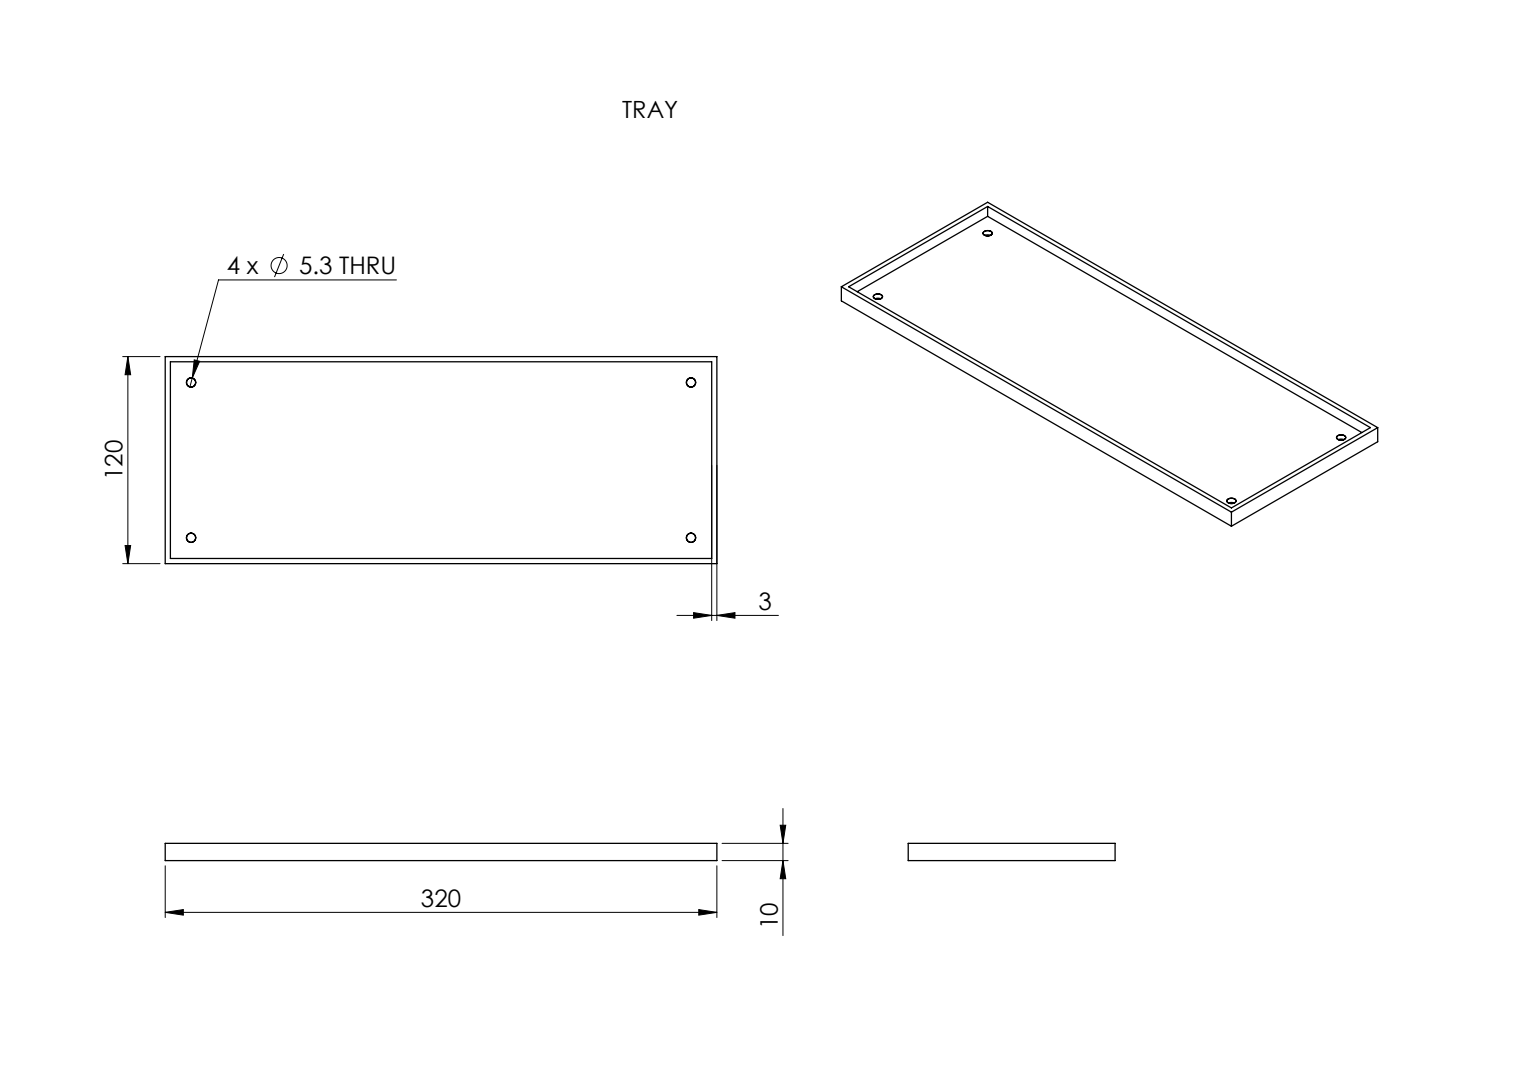
ISO-10303-21;
HEADER;
FILE_DESCRIPTION (('STEP AP214'),
    '1' );
FILE_NAME ('tray.step',
    '2026-10-23T15:04:32',
    ( '' ),
    ( '' ),
    'SwSTEP 2.0',
    'SolidWorks 2026',
    '' );
FILE_SCHEMA (( 'AUTOMOTIVE_DESIGN' ));
ENDSEC;

DATA;
#6=ORIENTED_EDGE ( 'NONE', *, *, #567, .F. ) ;
#7=CARTESIAN_POINT ( 'NONE',  ( 145.0000000000000284, 2.993649167310367343, -47.64999999999998437 ) ) ;
#14=ORIENTED_EDGE ( 'NONE', *, *, #1898, .T. ) ;
#15=FACE_OUTER_BOUND ( 'NONE', #510, .T. ) ;
#18=CIRCLE ( 'NONE', #321, 2.700000000000001066 ) ;
#19=ORIENTED_EDGE ( 'NONE', *, *, #1395, .T. ) ;
#21=CARTESIAN_POINT ( 'NONE',  ( 157.0000000000000000, 10.00000000000000000, 3.631354476378115974E-14 ) ) ;
#24=ORIENTED_EDGE ( 'NONE', *, *, #1544, .T. ) ;
#25=CARTESIAN_POINT ( 'NONE',  ( -145.0000000000000284, 3.000000000000000000, -45.00000000000000000 ) ) ;
#26=DIRECTION ( 'NONE',  ( -0.000000000000000000, 1.000000000000000000, -0.000000000000000000 ) ) ;
#27=CYLINDRICAL_SURFACE ( 'NONE', #1694, 2.649999999999985700 ) ;
#30=AXIS2_PLACEMENT_3D ( 'NONE', #971, #1660, #79 ) ;
#31=CIRCLE ( 'NONE', #984, 2.649999999999985700 ) ;
#35=ORIENTED_EDGE ( 'NONE', *, *, #686, .F. ) ;
#36=CYLINDRICAL_SURFACE ( 'NONE', #640, 2.649999999999985700 ) ;
#39=DIRECTION ( 'NONE',  ( -6.123233995736766036E-17, 1.000000000000000000, -0.000000000000000000 ) ) ;
#44=VERTEX_POINT ( 'NONE', #1009 ) ;
#46=CARTESIAN_POINT ( 'NONE',  ( 160.0000000000000000, 0.000000000000000000, -60.00000000000000000 ) ) ;
#47=CARTESIAN_POINT ( 'NONE',  ( 160.0000000000000000, 10.00000000000000000, -60.00000000000000000 ) ) ;
#48=PLANE ( 'NONE',  #876 ) ;
#49=ORIENTED_EDGE ( 'NONE', *, *, #111, .T. ) ;
#50=DIRECTION ( 'NONE',  ( -0.000000000000000000, 1.000000000000000000, -0.000000000000000000 ) ) ;
#51=AXIS2_PLACEMENT_3D ( 'NONE', #1269, #57, #1759 ) ;
#57=DIRECTION ( 'NONE',  ( 6.123233995736766036E-17, -1.000000000000000000, 0.000000000000000000 ) ) ;
#59=DIRECTION ( 'NONE',  ( -0.000000000000000000, -1.000000000000000000, -0.000000000000000000 ) ) ;
#60=VERTEX_POINT ( 'NONE', #817 ) ;
#66=ADVANCED_FACE ( 'NONE', ( #1330, #2016 ), #1163, .F. ) ;
#67=AXIS2_PLACEMENT_3D ( 'NONE', #1690, #1835, #1322 ) ;
#69=DIRECTION ( 'NONE',  ( -1.000000000000000000, 0.000000000000000000, -0.000000000000000000 ) ) ;
#70=LINE ( 'NONE', #2132, #1985 ) ;
#71=AXIS2_PLACEMENT_3D ( 'NONE', #2013, #995, #1317 ) ;
#73=CARTESIAN_POINT ( 'NONE',  ( 145.0000000000000284, 2.993649167310367343, -45.00000000000000000 ) ) ;
#77=DIRECTION ( 'NONE',  ( 0.000000000000000000, 0.000000000000000000, -1.000000000000000000 ) ) ;
#79=DIRECTION ( 'NONE',  ( 1.000000000000000000, 0.000000000000000000, 0.000000000000000000 ) ) ;
#82=FACE_OUTER_BOUND ( 'NONE', #1924, .T. ) ;
#88=VECTOR ( 'NONE', #539, 1000.000000000000000 ) ;
#90=CARTESIAN_POINT ( 'NONE',  ( -157.0000000000000284, 10.00000000000000000, 57.00000000000000711 ) ) ;
#93=( LENGTH_UNIT ( ) NAMED_UNIT ( * ) SI_UNIT ( .MILLI., .METRE. ) );
#100=ORIENTED_EDGE ( 'NONE', *, *, #520, .T. ) ;
#102=CARTESIAN_POINT ( 'NONE',  ( -160.0000000000000000, 10.00000000000000000, -56.99999999999997868 ) ) ;
#103=AXIS2_PLACEMENT_3D ( 'NONE', #1867, #1367, #311 ) ;
#109=PLANE ( 'NONE',  #1726 ) ;
#111=EDGE_CURVE ( 'NONE', #1963, #60, #1752, .T. ) ;
#114=DIRECTION ( 'NONE',  ( 1.000000000000000000, 0.000000000000000000, -4.336808689942017736E-17 ) ) ;
#117=( GEOMETRIC_REPRESENTATION_CONTEXT ( 3 ) GLOBAL_UNCERTAINTY_ASSIGNED_CONTEXT ( ( #842 ) ) GLOBAL_UNIT_ASSIGNED_CONTEXT ( ( #1606, #589, #1445 ) ) REPRESENTATION_CONTEXT ( 'NONE', 'WORKASPACE' ) );
#119=CARTESIAN_POINT ( 'NONE',  ( -145.0000000000000284, 0.000000000000000000, 42.35000000000001563 ) ) ;
#120=CARTESIAN_POINT ( 'NONE',  ( 156.9999999999999716, 3.000000000000000000, 57.00000000000000711 ) ) ;
#121=EDGE_CURVE ( 'NONE', #1963, #166, #205, .T. ) ;
#128=DIRECTION ( 'NONE',  ( 1.000000000000000000, 0.000000000000000000, 0.000000000000000000 ) ) ;
#129=AXIS2_PLACEMENT_3D ( 'NONE', #1889, #358, #1728 ) ;
#131=FILL_AREA_STYLE_COLOUR ( '', #721 ) ;
#135=EDGE_CURVE ( 'NONE', #1670, #1316, #2046, .T. ) ;
#137=CARTESIAN_POINT ( 'NONE',  ( 145.0000000000000284, 3.000000000000002665, -45.00000000000000000 ) ) ;
#142=DIRECTION ( 'NONE',  ( 0.000000000000000000, 0.000000000000000000, -1.000000000000000000 ) ) ;
#146=ADVANCED_FACE ( 'NONE', ( #978 ), #2193, .F. ) ;
#148=ORIENTED_EDGE ( 'NONE', *, *, #1970, .F. ) ;
#151=ORIENTED_EDGE ( 'NONE', *, *, #1176, .T. ) ;
#152=VECTOR ( 'NONE', #723, 1000.000000000000000 ) ;
#154=FACE_OUTER_BOUND ( 'NONE', #1037, .T. ) ;
#158=ORIENTED_EDGE ( 'NONE', *, *, #281, .T. ) ;
#159=DIRECTION ( 'NONE',  ( 0.000000000000000000, -1.000000000000000000, 0.000000000000000000 ) ) ;
#160=CARTESIAN_POINT ( 'NONE',  ( -145.0000000000000284, 3.000000000000001776, -47.70000000000000284 ) ) ;
#166=VERTEX_POINT ( 'NONE', #1403 ) ;
#167=ORIENTED_EDGE ( 'NONE', *, *, #1762, .T. ) ;
#168=VECTOR ( 'NONE', #1538, 1000.000000000000000 ) ;
#169=CYLINDRICAL_SURFACE ( 'NONE', #1242, 2.649999999999985700 ) ;
#170=CARTESIAN_POINT ( 'NONE',  ( -157.0000000000000000, 10.00000000000000000, -3.631354476378115974E-14 ) ) ;
#171=ADVANCED_FACE ( 'NONE', ( #512 ), #704, .T. ) ;
#176=ORIENTED_EDGE ( 'NONE', *, *, #1772, .T. ) ;
#177=AXIS2_PLACEMENT_3D ( 'NONE', #1608, #438, #449 ) ;
#178=ORIENTED_EDGE ( 'NONE', *, *, #684, .F. ) ;
#179=FACE_OUTER_BOUND ( 'NONE', #272, .T. ) ;
#181=CARTESIAN_POINT ( 'NONE',  ( -160.0000000000000284, 0.000000000000000000, 60.00000000000001421 ) ) ;
#182=AXIS2_PLACEMENT_3D ( 'NONE', #632, #455, #1006 ) ;
#186=EDGE_CURVE ( 'NONE', #1465, #166, #1054, .T. ) ;
#197=EDGE_CURVE ( 'NONE', #1465, #610, #889, .T. ) ;
#199=LINE ( 'NONE', #1861, #548 ) ;
#202=CARTESIAN_POINT ( 'NONE',  ( 145.0000000000000284, 3.000000000000001776, -47.70000000000000284 ) ) ;
#204=ORIENTED_EDGE ( 'NONE', *, *, #1315, .F. ) ;
#205=CIRCLE ( 'NONE', #1463, 2.649999999999985700 ) ;
#210=CARTESIAN_POINT ( 'NONE',  ( -160.0000000000000000, 10.00000000000000000, -59.99999999999998579 ) ) ;
#211=DIRECTION ( 'NONE',  ( 0.000000000000000000, 0.000000000000000000, -1.000000000000000000 ) ) ;
#214=EDGE_LOOP ( 'NONE', ( #762, #945, #1306, #1209 ) ) ;
#216=VERTEX_POINT ( 'NONE', #7 ) ;
#217=FACE_OUTER_BOUND ( 'NONE', #1185, .T. ) ;
#218=CARTESIAN_POINT ( 'NONE',  ( 160.0000000000000000, 10.00000000000000000, -60.00000000000000000 ) ) ;
#219=DIRECTION ( 'NONE',  ( 4.336808689942017736E-17, -0.000000000000000000, 1.000000000000000000 ) ) ;
#223=DIRECTION ( 'NONE',  ( -1.000000000000000000, -6.123233995736766036E-17, -0.000000000000000000 ) ) ;
#225=ORIENTED_EDGE ( 'NONE', *, *, #1492, .F. ) ;
#227=CIRCLE ( 'NONE', #385, 2.700000000000001066 ) ;
#230=CARTESIAN_POINT ( 'NONE',  ( -160.0000000000000284, 10.00000000000000000, 60.00000000000001421 ) ) ;
#231=CARTESIAN_POINT ( 'NONE',  ( -2.471980953266949321E-15, 3.000000000000000000, -56.99999999999998579 ) ) ;
#234=ORIENTED_EDGE ( 'NONE', *, *, #1075, .T. ) ;
#235=ORIENTED_EDGE ( 'NONE', *, *, #197, .F. ) ;
#238=FACE_OUTER_BOUND ( 'NONE', #1600, .T. ) ;
#240=VERTEX_POINT ( 'NONE', #1377 ) ;
#242=AXIS2_PLACEMENT_3D ( 'NONE', #919, #223, #2104 ) ;
#243=DIRECTION ( 'NONE',  ( -1.000000000000000000, 0.000000000000000000, 4.336808689942017736E-17 ) ) ;
#246=ADVANCED_FACE ( 'NONE', ( #1385 ), #1674, .T. ) ;
#250=VECTOR ( 'NONE', #1166, 1000.000000000000000 ) ;
#251=ORIENTED_EDGE ( 'NONE', *, *, #1272, .F. ) ;
#252=DIRECTION ( 'NONE',  ( -0.000000000000000000, 1.000000000000000000, -0.000000000000000000 ) ) ;
#253=CARTESIAN_POINT ( 'NONE',  ( -145.0000000000000284, 3.000000000000002665, 45.00000000000000000 ) ) ;
#256=VERTEX_POINT ( 'NONE', #1555 ) ;
#258=DIRECTION ( 'NONE',  ( -0.000000000000000000, 1.000000000000000000, -0.000000000000000000 ) ) ;
#259=ORIENTED_EDGE ( 'NONE', *, *, #781, .F. ) ;
#260=DIRECTION ( 'NONE',  ( -1.000000000000000000, -6.123233995736766036E-17, -0.000000000000000000 ) ) ;
#261=SHAPE_REPRESENTATION ( 'tray', ( #30 ), #1049 ) ;
#262=DIRECTION ( 'NONE',  ( 0.000000000000000000, -1.000000000000000000, 0.000000000000000000 ) ) ;
#263=LINE ( 'NONE', #90, #1184 ) ;
#266=EDGE_CURVE ( 'NONE', #1421, #653, #1916, .T. ) ;
#267=VERTEX_POINT ( 'NONE', #707 ) ;
#272=EDGE_LOOP ( 'NONE', ( #1135, #854, #1328, #1129 ) ) ;
#273=CARTESIAN_POINT ( 'NONE',  ( 145.0000000000000284, 2.800000000000000266, -45.00000000000000000 ) ) ;
#276=FACE_OUTER_BOUND ( 'NONE', #1110, .T. ) ;
#279=PRODUCT_DEFINITION_SHAPE ( 'NONE', 'NONE',  #1642 ) ;
#281=EDGE_CURVE ( 'NONE', #240, #1735, #1638, .T. ) ;
#282=ORIENTED_EDGE ( 'NONE', *, *, #559, .F. ) ;
#287=ADVANCED_FACE ( 'NONE', ( #15 ), #36, .F. ) ;
#298=AXIS2_PLACEMENT_3D ( 'NONE', #2174, #1189, #2020 ) ;
#305=ADVANCED_FACE ( 'NONE', ( #1736 ), #169, .F. ) ;
#307=( NAMED_UNIT ( * ) PLANE_ANGLE_UNIT ( ) SI_UNIT ( $, .RADIAN. ) );
#308=ORIENTED_EDGE ( 'NONE', *, *, #734, .F. ) ;
#311=DIRECTION ( 'NONE',  ( 0.000000000000000000, -1.000000000000000000, 0.000000000000000000 ) ) ;
#315=DIRECTION ( 'NONE',  ( -6.123233995736766036E-17, 1.000000000000000000, -0.000000000000000000 ) ) ;
#317=CARTESIAN_POINT ( 'NONE',  ( -145.0000000000000284, 0.000000000000000000, -45.00000000000000000 ) ) ;
#321=AXIS2_PLACEMENT_3D ( 'NONE', #1424, #399, #1951 ) ;
#323=DIRECTION ( 'NONE',  ( -0.000000000000000000, 1.000000000000000000, -0.000000000000000000 ) ) ;
#326=DIRECTION ( 'NONE',  ( 6.123233995736766036E-17, -1.000000000000000000, 0.000000000000000000 ) ) ;
#330=DIRECTION ( 'NONE',  ( 2.312964634635742957E-16, 0.000000000000000000, -1.000000000000000000 ) ) ;
#332=ORIENTED_EDGE ( 'NONE', *, *, #1547, .T. ) ;
#334=EDGE_CURVE ( 'NONE', #396, #60, #18, .T. ) ;
#336=MECHANICAL_DESIGN_GEOMETRIC_PRESENTATION_REPRESENTATION('',(#1119),#1476);
#337=ORIENTED_EDGE ( 'NONE', *, *, #2208, .F. ) ;
#339=CARTESIAN_POINT ( 'NONE',  ( -157.0000000000000284, 3.000000000000000000, 57.00000000000000711 ) ) ;
#341=STYLED_ITEM('',(#2247),#969);
#343=EDGE_LOOP ( 'NONE', ( #996, #736, #151, #176 ) ) ;
#344=VERTEX_POINT ( 'NONE', #572 ) ;
#345=ADVANCED_FACE ( 'NONE', ( #1256 ), #564, .T. ) ;
#346=DIRECTION ( 'NONE',  ( 0.000000000000000000, 0.000000000000000000, 1.000000000000000000 ) ) ;
#348=UNCERTAINTY_MEASURE_WITH_UNIT (LENGTH_MEASURE( 1.000000000000000082E-05 ), #93, 'distance_accuracy_value', 'NONE');
#350=DIRECTION ( 'NONE',  ( 1.000000000000000000, 0.000000000000000000, 0.000000000000000000 ) ) ;
#351=EDGE_LOOP ( 'NONE', ( #436, #2147 ) ) ;
#352=ADVANCED_FACE ( 'NONE', ( #217 ), #1742, .T. ) ;
#353=VERTEX_POINT ( 'NONE', #46 ) ;
#355=AXIS2_PLACEMENT_3D ( 'NONE', #1066, #872, #1906 ) ;
#358=DIRECTION ( 'NONE',  ( 6.123233995736766036E-17, -1.000000000000000000, 0.000000000000000000 ) ) ;
#365=DIRECTION ( 'NONE',  ( 0.000000000000000000, 0.000000000000000000, -1.000000000000000000 ) ) ;
#375=EDGE_LOOP ( 'NONE', ( #1502, #922, #259, #2033 ) ) ;
#377=DIRECTION ( 'NONE',  ( 0.000000000000000000, -1.000000000000000000, 0.000000000000000000 ) ) ;
#379=EDGE_LOOP ( 'NONE', ( #1466, #491 ) ) ;
#381=EDGE_CURVE ( 'NONE', #344, #473, #457, .T. ) ;
#385=AXIS2_PLACEMENT_3D ( 'NONE', #1320, #1495, #1483 ) ;
#386=ORIENTED_EDGE ( 'NONE', *, *, #744, .T. ) ;
#387=ORIENTED_EDGE ( 'NONE', *, *, #767, .F. ) ;
#389=CYLINDRICAL_SURFACE ( 'NONE', #1669, 2.649999999999985700 ) ;
#390=PLANE ( 'NONE',  #760 ) ;
#392=CARTESIAN_POINT ( 'NONE',  ( -160.0000000000000284, 10.00000000000000000, 60.00000000000001421 ) ) ;
#396=VERTEX_POINT ( 'NONE', #2094 ) ;
#397=VECTOR ( 'NONE', #1100, 1000.000000000000000 ) ;
#399=DIRECTION ( 'NONE',  ( -6.123233995736766036E-17, 1.000000000000000000, -0.000000000000000000 ) ) ;
#408=DIRECTION ( 'NONE',  ( 0.000000000000000000, 0.000000000000000000, -1.000000000000000000 ) ) ;
#409=DIRECTION ( 'NONE',  ( -0.000000000000000000, -1.000000000000000000, -0.000000000000000000 ) ) ;
#412=CARTESIAN_POINT ( 'NONE',  ( -160.0000000000000284, 0.000000000000000000, 60.00000000000001421 ) ) ;
#415=VERTEX_POINT ( 'NONE', #1060 ) ;
#417=EDGE_LOOP ( 'NONE', ( #282, #2155, #528, #1458 ) ) ;
#418=VECTOR ( 'NONE', #409, 1000.000000000000000 ) ;
#419=DIRECTION ( 'NONE',  ( 0.000000000000000000, 0.000000000000000000, 1.000000000000000000 ) ) ;
#420=DIRECTION ( 'NONE',  ( 0.000000000000000000, -1.000000000000000000, 0.000000000000000000 ) ) ;
#423=ADVANCED_FACE ( 'NONE', ( #1755 ), #626, .F. ) ;
#426=FACE_BOUND ( 'NONE', #2181, .T. ) ;
#428=( LENGTH_UNIT ( ) NAMED_UNIT ( * ) SI_UNIT ( .MILLI., .METRE. ) );
#429=VECTOR ( 'NONE', #1167, 1000.000000000000000 ) ;
#433=DIRECTION ( 'NONE',  ( 1.000000000000000000, 0.000000000000000000, 0.000000000000000000 ) ) ;
#434=DIRECTION ( 'NONE',  ( 0.000000000000000000, 0.000000000000000000, -1.000000000000000000 ) ) ;
#436=ORIENTED_EDGE ( 'NONE', *, *, #2067, .F. ) ;
#437=AXIS2_PLACEMENT_3D ( 'NONE', #747, #702, #1251 ) ;
#438=DIRECTION ( 'NONE',  ( 0.000000000000000000, -1.000000000000000000, 0.000000000000000000 ) ) ;
#441=AXIS2_PLACEMENT_3D ( 'NONE', #484, #315, #1178 ) ;
#443=CARTESIAN_POINT ( 'NONE',  ( 145.0000000000000284, 2.993649167310367343, -42.35000000000001563 ) ) ;
#448=CARTESIAN_POINT ( 'NONE',  ( -145.0000000000000284, 3.000000000000000000, 45.00000000000000000 ) ) ;
#449=DIRECTION ( 'NONE',  ( 0.000000000000000000, 0.000000000000000000, -1.000000000000000000 ) ) ;
#455=DIRECTION ( 'NONE',  ( 1.000000000000000000, 6.123233995736766036E-17, -1.224646799147353207E-16 ) ) ;
#457=LINE ( 'NONE', #1731, #1139 ) ;
#458=CARTESIAN_POINT ( 'NONE',  ( 145.0000000000000284, 2.993649167310367343, -45.00000000000000000 ) ) ;
#461=VECTOR ( 'NONE', #1047, 1000.000000000000000 ) ;
#465=ORIENTED_EDGE ( 'NONE', *, *, #819, .F. ) ;
#467=EDGE_CURVE ( 'NONE', #486, #1704, #896, .T. ) ;
#473=VERTEX_POINT ( 'NONE', #1228 ) ;
#482=EDGE_CURVE ( 'NONE', #486, #1700, #1469, .T. ) ;
#484=CARTESIAN_POINT ( 'NONE',  ( 145.0000000000000284, 3.000000000000002665, 45.00000000000000000 ) ) ;
#486=VERTEX_POINT ( 'NONE', #1921 ) ;
#487=CARTESIAN_POINT ( 'NONE',  ( -160.0000000000000284, 10.00000000000000000, 60.00000000000001421 ) ) ;
#491=ORIENTED_EDGE ( 'NONE', *, *, #1236, .F. ) ;
#494=CARTESIAN_POINT ( 'NONE',  ( -160.0000000000000284, 10.00000000000000000, 60.00000000000001421 ) ) ;
#497=EDGE_LOOP ( 'NONE', ( #1053, #1791, #14, #2049 ) ) ;
#498=ORIENTED_EDGE ( 'NONE', *, *, #929, .F. ) ;
#501=VECTOR ( 'NONE', #330, 1000.000000000000000 ) ;
#507=CIRCLE ( 'NONE', #242, 0.2000000000000000944 ) ;
#509=EDGE_CURVE ( 'NONE', #216, #1444, #1194, .T. ) ;
#510=EDGE_LOOP ( 'NONE', ( #1989, #1715, #2217, #1147 ) ) ;
#512=FACE_OUTER_BOUND ( 'NONE', #1696, .T. ) ;
#513=CARTESIAN_POINT ( 'NONE',  ( -145.0000000000000284, 2.800000000000000266, -47.70000000000000284 ) ) ;
#517=VECTOR ( 'NONE', #953, 1000.000000000000000 ) ;
#520=EDGE_CURVE ( 'NONE', #665, #473, #1798, .T. ) ;
#522=EDGE_CURVE ( 'NONE', #1661, #415, #1521, .T. ) ;
#523=ORIENTED_EDGE ( 'NONE', *, *, #197, .T. ) ;
#527=VECTOR ( 'NONE', #1737, 1000.000000000000000 ) ;
#528=ORIENTED_EDGE ( 'NONE', *, *, #186, .T. ) ;
#529=CARTESIAN_POINT ( 'NONE',  ( -145.0000000000000284, 0.000000000000000000, 45.00000000000000000 ) ) ;
#530=DIRECTION ( 'NONE',  ( 1.000000000000000000, 0.000000000000000000, 0.000000000000000000 ) ) ;
#539=DIRECTION ( 'NONE',  ( -2.312964634635742957E-16, 0.000000000000000000, 1.000000000000000000 ) ) ;
#542=DIRECTION ( 'NONE',  ( 0.000000000000000000, -1.000000000000000000, 0.000000000000000000 ) ) ;
#543=EDGE_CURVE ( 'NONE', #1735, #1188, #1860, .T. ) ;
#548=VECTOR ( 'NONE', #1691, 1000.000000000000000 ) ;
#552=CARTESIAN_POINT ( 'NONE',  ( -145.0000000000000284, 2.993649167310367343, -45.00000000000000000 ) ) ;
#559=EDGE_CURVE ( 'NONE', #610, #1963, #1824, .T. ) ;
#560=ORIENTED_EDGE ( 'NONE', *, *, #686, .T. ) ;
#564=TOROIDAL_SURFACE ( 'NONE', #51, 2.700000000000000622, 0.2000000000000000111 ) ;
#567=EDGE_CURVE ( 'NONE', #1735, #240, #1938, .T. ) ;
#571=EDGE_LOOP ( 'NONE', ( #498, #1915, #1230, #1366 ) ) ;
#572=CARTESIAN_POINT ( 'NONE',  ( -145.0000000000000284, 0.000000000000000000, -42.35000000000001563 ) ) ;
#574=CARTESIAN_POINT ( 'NONE',  ( -145.0000000000000284, 2.993649167310367343, 42.35000000000001563 ) ) ;
#577=LINE ( 'NONE', #231, #1370 ) ;
#580=EDGE_CURVE ( 'NONE', #898, #1725, #31, .T. ) ;
#581=VECTOR ( 'NONE', #59, 1000.000000000000000 ) ;
#582=CARTESIAN_POINT ( 'NONE',  ( -145.0000000000000284, 2.993649167310367343, -45.00000000000000000 ) ) ;
#583=AXIS2_PLACEMENT_3D ( 'NONE', #756, #260, #1459 ) ;
#589=( NAMED_UNIT ( * ) PLANE_ANGLE_UNIT ( ) SI_UNIT ( $, .RADIAN. ) );
#590=FACE_BOUND ( 'NONE', #2014, .T. ) ;
#592=ORIENTED_EDGE ( 'NONE', *, *, #482, .T. ) ;
#594=AXIS2_PLACEMENT_3D ( 'NONE', #1603, #1291, #433 ) ;
#595=CYLINDRICAL_SURFACE ( 'NONE', #1464, 2.649999999999985700 ) ;
#598=ORIENTED_EDGE ( 'NONE', *, *, #111, .F. ) ;
#603=DIRECTION ( 'NONE',  ( 1.000000000000000000, 0.000000000000000000, 0.000000000000000000 ) ) ;
#606=ORIENTED_EDGE ( 'NONE', *, *, #850, .F. ) ;
#610=VERTEX_POINT ( 'NONE', #119 ) ;
#613=DIRECTION ( 'NONE',  ( 0.000000000000000000, 0.000000000000000000, -1.000000000000000000 ) ) ;
#619=ORIENTED_EDGE ( 'NONE', *, *, #914, .T. ) ;
#621=VECTOR ( 'NONE', #683, 1000.000000000000000 ) ;
#626=PLANE ( 'NONE',  #785 ) ;
#631=ORIENTED_EDGE ( 'NONE', *, *, #1970, .T. ) ;
#632=CARTESIAN_POINT ( 'NONE',  ( 145.0000000000000284, 2.800000000000000266, -42.29999999999999716 ) ) ;
#635=CIRCLE ( 'NONE', #1354, 2.700000000000001066 ) ;
#638=CARTESIAN_POINT ( 'NONE',  ( -145.0000000000000284, 3.000000000000000000, 42.35000000000001563 ) ) ;
#640=AXIS2_PLACEMENT_3D ( 'NONE', #2075, #1219, #346 ) ;
#645=EDGE_CURVE ( 'NONE', #1390, #267, #657, .T. ) ;
#650=CARTESIAN_POINT ( 'NONE',  ( 145.0000000000000284, 3.000000000000000000, 42.35000000000001563 ) ) ;
#653=VERTEX_POINT ( 'NONE', #2223 ) ;
#654=FACE_OUTER_BOUND ( 'NONE', #571, .T. ) ;
#656=PRODUCT_DEFINITION_FORMATION_WITH_SPECIFIED_SOURCE ( 'ANY', '', #1962, .NOT_KNOWN. ) ;
#657=CIRCLE ( 'NONE', #298, 2.700000000000001066 ) ;
#658=DIRECTION ( 'NONE',  ( 6.123233995736766036E-17, -1.000000000000000000, 0.000000000000000000 ) ) ;
#659=CIRCLE ( 'NONE', #2087, 2.700000000000001066 ) ;
#665=VERTEX_POINT ( 'NONE', #1701 ) ;
#667=ORIENTED_EDGE ( 'NONE', *, *, #1241, .T. ) ;
#668=DIRECTION ( 'NONE',  ( -6.123233995736766036E-17, 1.000000000000000000, -0.000000000000000000 ) ) ;
#669=DIRECTION ( 'NONE',  ( 4.336808689942017736E-17, -0.000000000000000000, 1.000000000000000000 ) ) ;
#674=DIRECTION ( 'NONE',  ( 0.000000000000000000, 0.000000000000000000, 1.000000000000000000 ) ) ;
#683=DIRECTION ( 'NONE',  ( -1.000000000000000000, -0.000000000000000000, 4.336808689942017736E-17 ) ) ;
#684=EDGE_CURVE ( 'NONE', #267, #1390, #942, .T. ) ;
#686=EDGE_CURVE ( 'NONE', #1439, #835, #831, .T. ) ;
#689=CARTESIAN_POINT ( 'NONE',  ( -145.0000000000000284, 3.000000000000000000, 47.64999999999998437 ) ) ;
#693=CIRCLE ( 'NONE', #583, 0.2000000000000000944 ) ;
#694=VERTEX_POINT ( 'NONE', #339 ) ;
#695=ORIENTED_EDGE ( 'NONE', *, *, #850, .T. ) ;
#697=DIRECTION ( 'NONE',  ( 0.000000000000000000, -1.000000000000000000, 0.000000000000000000 ) ) ;
#701=CIRCLE ( 'NONE', #816, 2.649999999999985700 ) ;
#702=DIRECTION ( 'NONE',  ( 1.000000000000000000, -0.000000000000000000, 2.312964634635742957E-16 ) ) ;
#704=TOROIDAL_SURFACE ( 'NONE', #859, 2.700000000000000622, 0.2000000000000000111 ) ;
#707=CARTESIAN_POINT ( 'NONE',  ( 145.0000000000000284, 3.000000000000001776, 42.29999999999999716 ) ) ;
#708=FACE_OUTER_BOUND ( 'NONE', #1170, .T. ) ;
#712=VECTOR ( 'NONE', #893, 1000.000000000000000 ) ;
#714=AXIS2_PLACEMENT_3D ( 'NONE', #1093, #262, #1427 ) ;
#716=ORIENTED_EDGE ( 'NONE', *, *, #580, .F. ) ;
#717=DIRECTION ( 'NONE',  ( 6.123233995736766036E-17, -1.000000000000000000, 0.000000000000000000 ) ) ;
#718=CARTESIAN_POINT ( 'NONE',  ( -145.0000000000000284, 3.000000000000002665, -45.00000000000000000 ) ) ;
#721=COLOUR_RGB ( '',0.8941176470588234615, 0.8941176470588234615, 0.8941176470588234615 ) ;
#723=DIRECTION ( 'NONE',  ( 0.000000000000000000, -1.000000000000000000, 0.000000000000000000 ) ) ;
#724=MECHANICAL_DESIGN_GEOMETRIC_PRESENTATION_REPRESENTATION('',(#341),#117);
#726=TOROIDAL_SURFACE ( 'NONE', #2121, 2.700000000000000622, 0.2000000000000000111 ) ;
#732=FACE_OUTER_BOUND ( 'NONE', #375, .T. ) ;
#733=CYLINDRICAL_SURFACE ( 'NONE', #1554, 2.649999999999985700 ) ;
#734=EDGE_CURVE ( 'NONE', #610, #1465, #1834, .T. ) ;
#736=ORIENTED_EDGE ( 'NONE', *, *, #266, .F. ) ;
#744=EDGE_CURVE ( 'NONE', #166, #1963, #2116, .T. ) ;
#745=LINE ( 'NONE', #954, #2113 ) ;
#747=CARTESIAN_POINT ( 'NONE',  ( -157.0000000000000284, 10.00000000000000000, 60.00000000000001421 ) ) ;
#751=ORIENTED_EDGE ( 'NONE', *, *, #543, .F. ) ;
#756=CARTESIAN_POINT ( 'NONE',  ( 145.0000000000000284, 2.800000000000000266, 42.29999999999999716 ) ) ;
#759=VECTOR ( 'NONE', #1013, 1000.000000000000000 ) ;
#760=AXIS2_PLACEMENT_3D ( 'NONE', #1426, #219, #779 ) ;
#762=ORIENTED_EDGE ( 'NONE', *, *, #1790, .T. ) ;
#767=EDGE_CURVE ( 'NONE', #1725, #1444, #1884, .T. ) ;
#768=DIRECTION ( 'NONE',  ( 1.000000000000000000, 0.000000000000000000, 0.000000000000000000 ) ) ;
#770=DIRECTION ( 'NONE',  ( 2.312964634635742957E-16, 0.000000000000000000, -1.000000000000000000 ) ) ;
#772=LINE ( 'NONE', #1447, #1746 ) ;
#777=AXIS2_PLACEMENT_3D ( 'NONE', #102, #669, #114 ) ;
#779=DIRECTION ( 'NONE',  ( 1.000000000000000000, 0.000000000000000000, -4.336808689942017736E-17 ) ) ;
#780=ORIENTED_EDGE ( 'NONE', *, *, #1422, .T. ) ;
#781=EDGE_CURVE ( 'NONE', #1255, #1661, #1741, .T. ) ;
#783=EDGE_LOOP ( 'NONE', ( #1396, #1637, #1789, #387 ) ) ;
#785=AXIS2_PLACEMENT_3D ( 'NONE', #2159, #1114, #1630 ) ;
#787=DIRECTION ( 'NONE',  ( 0.000000000000000000, -1.000000000000000000, 0.000000000000000000 ) ) ;
#792=ORIENTED_EDGE ( 'NONE', *, *, #910, .F. ) ;
#800=SHAPE_DEFINITION_REPRESENTATION ( #279, #261 ) ;
#802=EDGE_LOOP ( 'NONE', ( #2028, #962, #952, #2198 ) ) ;
#808=DIRECTION ( 'NONE',  ( 1.000000000000000000, 0.000000000000000000, 0.000000000000000000 ) ) ;
#812=( NAMED_UNIT ( * ) SI_UNIT ( $, .STERADIAN. ) SOLID_ANGLE_UNIT ( ) );
#816=AXIS2_PLACEMENT_3D ( 'NONE', #458, #980, #808 ) ;
#817=CARTESIAN_POINT ( 'NONE',  ( -145.0000000000000284, 3.000000000000001776, 42.29999999999999716 ) ) ;
#819=EDGE_CURVE ( 'NONE', #1531, #665, #1586, .T. ) ;
#826=CYLINDRICAL_SURFACE ( 'NONE', #2161, 2.649999999999985700 ) ;
#827=ORIENTED_EDGE ( 'NONE', *, *, #543, .T. ) ;
#831=LINE ( 'NONE', #1510, #621 ) ;
#833=VERTEX_POINT ( 'NONE', #1379 ) ;
#835=VERTEX_POINT ( 'NONE', #1545 ) ;
#842=UNCERTAINTY_MEASURE_WITH_UNIT (LENGTH_MEASURE( 1.000000000000000082E-05 ), #1606, 'distance_accuracy_value', 'NONE');
#843=EDGE_LOOP ( 'NONE', ( #1841, #386, #49, #1490 ) ) ;
#845=DIRECTION ( 'NONE',  ( -0.000000000000000000, 1.000000000000000000, -0.000000000000000000 ) ) ;
#848=VERTEX_POINT ( 'NONE', #181 ) ;
#849=APPLICATION_CONTEXT ( 'automotive_design' ) ;
#850=EDGE_CURVE ( 'NONE', #473, #2218, #1945, .T. ) ;
#854=ORIENTED_EDGE ( 'NONE', *, *, #1315, .T. ) ;
#859=AXIS2_PLACEMENT_3D ( 'NONE', #1196, #717, #365 ) ;
#862=DIRECTION ( 'NONE',  ( -0.000000000000000000, 1.000000000000000000, -0.000000000000000000 ) ) ;
#864=ORIENTED_EDGE ( 'NONE', *, *, #1314, .T. ) ;
#865=CARTESIAN_POINT ( 'NONE',  ( -145.0000000000000284, 2.993649167310367343, 45.00000000000000000 ) ) ;
#872=DIRECTION ( 'NONE',  ( 6.123233995736766036E-17, -1.000000000000000000, 0.000000000000000000 ) ) ;
#875=AXIS2_PLACEMENT_3D ( 'NONE', #2226, #542, #211 ) ;
#876=AXIS2_PLACEMENT_3D ( 'NONE', #1434, #2120, #1782 ) ;
#877=DIRECTION ( 'NONE',  ( 1.000000000000000000, 6.123233995736766036E-17, -1.224646799147353207E-16 ) ) ;
#882=CARTESIAN_POINT ( 'NONE',  ( -157.0000000000000000, 10.00000000000000000, -56.99999999999997868 ) ) ;
#883=DIRECTION ( 'NONE',  ( 0.000000000000000000, 0.000000000000000000, 1.000000000000000000 ) ) ;
#886=DIRECTION ( 'NONE',  ( 2.312964634635742957E-16, 0.000000000000000000, -1.000000000000000000 ) ) ;
#889=CIRCLE ( 'NONE', #2219, 2.649999999999985700 ) ;
#893=DIRECTION ( 'NONE',  ( -0.000000000000000000, -1.000000000000000000, -0.000000000000000000 ) ) ;
#896=LINE ( 'NONE', #21, #2199 ) ;
#898=VERTEX_POINT ( 'NONE', #1249 ) ;
#902=DIRECTION ( 'NONE',  ( 6.123233995736766036E-17, -1.000000000000000000, 0.000000000000000000 ) ) ;
#904=DIRECTION ( 'NONE',  ( 6.123233995736766036E-17, -1.000000000000000000, 0.000000000000000000 ) ) ;
#910=EDGE_CURVE ( 'NONE', #1188, #267, #693, .T. ) ;
#913=FACE_BOUND ( 'NONE', #379, .T. ) ;
#914=EDGE_CURVE ( 'NONE', #256, #848, #1946, .T. ) ;
#919=CARTESIAN_POINT ( 'NONE',  ( 145.0000000000000284, 2.800000000000000266, -47.70000000000000284 ) ) ;
#922=ORIENTED_EDGE ( 'NONE', *, *, #522, .F. ) ;
#927=VECTOR ( 'NONE', #1972, 1000.000000000000000 ) ;
#929=EDGE_CURVE ( 'NONE', #1700, #44, #963, .T. ) ;
#931=EDGE_CURVE ( 'NONE', #166, #396, #2202, .T. ) ;
#934=LINE ( 'NONE', #2131, #397 ) ;
#936=DIRECTION ( 'NONE',  ( 6.123233995736766036E-17, -1.000000000000000000, 0.000000000000000000 ) ) ;
#941=ADVANCED_FACE ( 'NONE', ( #1982 ), #733, .F. ) ;
#942=CIRCLE ( 'NONE', #441, 2.700000000000001066 ) ;
#945=ORIENTED_EDGE ( 'NONE', *, *, #1314, .F. ) ;
#946=ADVANCED_FACE ( 'NONE', ( #1091 ), #1514, .T. ) ;
#952=ORIENTED_EDGE ( 'NONE', *, *, #1176, .F. ) ;
#953=DIRECTION ( 'NONE',  ( -2.312964634635742957E-16, -0.000000000000000000, 1.000000000000000000 ) ) ;
#954=CARTESIAN_POINT ( 'NONE',  ( 145.0000000000000284, 3.000000000000000000, -47.64999999999998437 ) ) ;
#956=EDGE_LOOP ( 'NONE', ( #158, #827, #204, #1550 ) ) ;
#962=ORIENTED_EDGE ( 'NONE', *, *, #1762, .F. ) ;
#963=LINE ( 'NONE', #1645, #1693 ) ;
#969=MANIFOLD_SOLID_BREP ( 'Cavity1', #2111 ) ;
#971=CARTESIAN_POINT ( 'NONE',  ( 0.000000000000000000, 0.000000000000000000, 0.000000000000000000 ) ) ;
#978=FACE_OUTER_BOUND ( 'NONE', #956, .T. ) ;
#980=DIRECTION ( 'NONE',  ( 6.123233995736766036E-17, -1.000000000000000000, 0.000000000000000000 ) ) ;
#981=DIRECTION ( 'NONE',  ( 0.000000000000000000, -1.000000000000000000, 0.000000000000000000 ) ) ;
#983=SHAPE_REPRESENTATION_RELATIONSHIP ( 'NONE' , 'NONE' ,  #261, #2138 ) ;
#984=AXIS2_PLACEMENT_3D ( 'NONE', #1496, #981, #1678 ) ;
#986=AXIS2_PLACEMENT_3D ( 'NONE', #2080, #877, #1388 ) ;
#987=ORIENTED_EDGE ( 'NONE', *, *, #559, .T. ) ;
#995=DIRECTION ( 'NONE',  ( -1.000000000000000000, 0.000000000000000000, -2.312964634635742957E-16 ) ) ;
#996=ORIENTED_EDGE ( 'NONE', *, *, #1197, .F. ) ;
#997=CIRCLE ( 'NONE', #594, 2.649999999999985700 ) ;
#1002=DIRECTION ( 'NONE',  ( -1.000000000000000000, 0.000000000000000000, 4.336808689942017736E-17 ) ) ;
#1006=DIRECTION ( 'NONE',  ( 0.000000000000000000, 0.000000000000000000, -1.000000000000000000 ) ) ;
#1009=CARTESIAN_POINT ( 'NONE',  ( 157.0000000000000000, 3.000000000000000000, -56.99999999999999289 ) ) ;
#1013=DIRECTION ( 'NONE',  ( -0.000000000000000000, 1.000000000000000000, -0.000000000000000000 ) ) ;
#1019=VECTOR ( 'NONE', #1025, 1000.000000000000000 ) ;
#1022=FACE_OUTER_BOUND ( 'NONE', #497, .T. ) ;
#1025=DIRECTION ( 'NONE',  ( -0.000000000000000000, 1.000000000000000000, -0.000000000000000000 ) ) ;
#1031=PLANE ( 'NONE',  #1955 ) ;
#1037=EDGE_LOOP ( 'NONE', ( #523, #987, #2096, #1277 ) ) ;
#1039=DIRECTION ( 'NONE',  ( 0.000000000000000000, 0.000000000000000000, 1.000000000000000000 ) ) ;
#1040=CARTESIAN_POINT ( 'NONE',  ( -160.0000000000000284, 10.00000000000000000, 60.00000000000001421 ) ) ;
#1041=CARTESIAN_POINT ( 'NONE',  ( -145.0000000000000284, 3.000000000000000000, -47.64999999999998437 ) ) ;
#1046=ORIENTED_EDGE ( 'NONE', *, *, #1900, .T. ) ;
#1047=DIRECTION ( 'NONE',  ( 0.000000000000000000, -1.000000000000000000, 0.000000000000000000 ) ) ;
#1048=CARTESIAN_POINT ( 'NONE',  ( -157.0000000000000000, 3.000000000000000000, -3.631354476378115974E-14 ) ) ;
#1049=( GEOMETRIC_REPRESENTATION_CONTEXT ( 3 ) GLOBAL_UNCERTAINTY_ASSIGNED_CONTEXT ( ( #348 ) ) GLOBAL_UNIT_ASSIGNED_CONTEXT ( ( #93, #307, #812 ) ) REPRESENTATION_CONTEXT ( 'NONE', 'WORKASPACE' ) );
#1053=ORIENTED_EDGE ( 'NONE', *, *, #1547, .F. ) ;
#1054=LINE ( 'NONE', #689, #168 ) ;
#1055=CARTESIAN_POINT ( 'NONE',  ( 145.0000000000000284, 2.993649167310367343, 42.35000000000001563 ) ) ;
#1060=CARTESIAN_POINT ( 'NONE',  ( 159.9999999999999716, 0.000000000000000000, 60.00000000000001421 ) ) ;
#1061=FACE_OUTER_BOUND ( 'NONE', #343, .T. ) ;
#1066=CARTESIAN_POINT ( 'NONE',  ( -145.0000000000000284, 2.800000000000000266, -45.00000000000000000 ) ) ;
#1070=CIRCLE ( 'NONE', #1365, 2.700000000000001066 ) ;
#1075=EDGE_CURVE ( 'NONE', #1159, #2218, #227, .T. ) ;
#1076=ORIENTED_EDGE ( 'NONE', *, *, #1588, .T. ) ;
#1083=AXIS2_PLACEMENT_3D ( 'NONE', #273, #1931, #1773 ) ;
#1086=ORIENTED_EDGE ( 'NONE', *, *, #645, .F. ) ;
#1087=ORIENTED_EDGE ( 'NONE', *, *, #1145, .T. ) ;
#1090=CARTESIAN_POINT ( 'NONE',  ( -145.0000000000000284, 2.800000000000000266, 45.00000000000000000 ) ) ;
#1091=FACE_OUTER_BOUND ( 'NONE', #1682, .T. ) ;
#1092=EDGE_CURVE ( 'NONE', #1188, #1663, #1635, .T. ) ;
#1093=CARTESIAN_POINT ( 'NONE',  ( 0.000000000000000000, 0.000000000000000000, 0.000000000000000000 ) ) ;
#1100=DIRECTION ( 'NONE',  ( -1.000000000000000000, -0.000000000000000000, 4.336808689942017736E-17 ) ) ;
#1106=LINE ( 'NONE', #1785, #927 ) ;
#1107=ADVANCED_FACE ( 'NONE', ( #1022 ), #1688, .T. ) ;
#1110=EDGE_LOOP ( 'NONE', ( #2079, #2004, #1371, #792 ) ) ;
#1111=ORIENTED_EDGE ( 'NONE', *, *, #135, .F. ) ;
#1113=FACE_BOUND ( 'NONE', #351, .T. ) ;
#1114=DIRECTION ( 'NONE',  ( -1.000000000000000000, 0.000000000000000000, -2.312964634635742957E-16 ) ) ;
#1117=FACE_OUTER_BOUND ( 'NONE', #2025, .T. ) ;
#1119=STYLED_ITEM ( 'NONE', ( #2188 ), #2138 ) ;
#1123=AXIS2_PLACEMENT_3D ( 'NONE', #230, #1750, #1628 ) ;
#1127=ORIENTED_EDGE ( 'NONE', *, *, #1923, .T. ) ;
#1129=ORIENTED_EDGE ( 'NONE', *, *, #684, .T. ) ;
#1135=ORIENTED_EDGE ( 'NONE', *, *, #1788, .F. ) ;
#1136=DIRECTION ( 'NONE',  ( 1.000000000000000000, -0.000000000000000000, 2.312964634635742957E-16 ) ) ;
#1139=VECTOR ( 'NONE', #258, 1000.000000000000000 ) ;
#1144=ORIENTED_EDGE ( 'NONE', *, *, #914, .F. ) ;
#1145=EDGE_CURVE ( 'NONE', #1444, #216, #701, .T. ) ;
#1146=CARTESIAN_POINT ( 'NONE',  ( -145.0000000000000284, 3.000000000000000000, -45.00000000000000000 ) ) ;
#1147=ORIENTED_EDGE ( 'NONE', *, *, #509, .F. ) ;
#1149=AXIS2_PLACEMENT_3D ( 'NONE', #1454, #420, #1270 ) ;
#1151=DIRECTION ( 'NONE',  ( 1.000000000000000000, 0.000000000000000000, 0.000000000000000000 ) ) ;
#1154=DIRECTION ( 'NONE',  ( 0.000000000000000000, 0.000000000000000000, -1.000000000000000000 ) ) ;
#1159=VERTEX_POINT ( 'NONE', #160 ) ;
#1163=PLANE ( 'NONE',  #1540 ) ;
#1166=DIRECTION ( 'NONE',  ( -0.000000000000000000, -1.000000000000000000, -0.000000000000000000 ) ) ;
#1167=DIRECTION ( 'NONE',  ( 1.000000000000000000, 0.000000000000000000, 0.000000000000000000 ) ) ;
#1170=EDGE_LOOP ( 'NONE', ( #1976, #1493, #167, #592 ) ) ;
#1172=ORIENTED_EDGE ( 'NONE', *, *, #520, .F. ) ;
#1176=EDGE_CURVE ( 'NONE', #1421, #833, #1907, .T. ) ;
#1178=DIRECTION ( 'NONE',  ( 0.000000000000000000, 0.000000000000000000, -1.000000000000000000 ) ) ;
#1184=VECTOR ( 'NONE', #787, 1000.000000000000000 ) ;
#1185=EDGE_LOOP ( 'NONE', ( #1512, #1326, #2170, #598 ) ) ;
#1188=VERTEX_POINT ( 'NONE', #1055 ) ;
#1189=DIRECTION ( 'NONE',  ( -6.123233995736766036E-17, 1.000000000000000000, -0.000000000000000000 ) ) ;
#1190=DIRECTION ( 'NONE',  ( 1.000000000000000000, 6.123233995736766036E-17, -1.224646799147353207E-16 ) ) ;
#1192=ORIENTED_EDGE ( 'NONE', *, *, #781, .T. ) ;
#1194=CIRCLE ( 'NONE', #1983, 2.649999999999985700 ) ;
#1195=VECTOR ( 'NONE', #1891, 1000.000000000000000 ) ;
#1196=CARTESIAN_POINT ( 'NONE',  ( 145.0000000000000284, 2.800000000000000266, -45.00000000000000000 ) ) ;
#1197=EDGE_CURVE ( 'NONE', #653, #694, #2090, .T. ) ;
#1199=PRODUCT_DEFINITION_CONTEXT ( 'detailed design', #1501, 'design' ) ;
#1203=ORIENTED_EDGE ( 'NONE', *, *, #135, .T. ) ;
#1204=DIRECTION ( 'NONE',  ( -0.000000000000000000, 1.000000000000000000, -0.000000000000000000 ) ) ;
#1205=CARTESIAN_POINT ( 'NONE',  ( 145.0000000000000284, 3.000000000000000000, -45.00000000000000000 ) ) ;
#1209=ORIENTED_EDGE ( 'NONE', *, *, #522, .T. ) ;
#1210=CIRCLE ( 'NONE', #1149, 2.649999999999985700 ) ;
#1214=ADVANCED_FACE ( 'NONE', ( #1233 ), #389, .F. ) ;
#1219=DIRECTION ( 'NONE',  ( -0.000000000000000000, 1.000000000000000000, -0.000000000000000000 ) ) ;
#1223=AXIS2_PLACEMENT_3D ( 'NONE', #582, #1666, #128 ) ;
#1227=DIRECTION ( 'NONE',  ( 1.000000000000000000, 0.000000000000000000, 0.000000000000000000 ) ) ;
#1228=CARTESIAN_POINT ( 'NONE',  ( -145.0000000000000284, 2.993649167310367343, -42.35000000000001563 ) ) ;
#1230=ORIENTED_EDGE ( 'NONE', *, *, #467, .T. ) ;
#1233=FACE_OUTER_BOUND ( 'NONE', #783, .T. ) ;
#1236=EDGE_CURVE ( 'NONE', #2218, #1159, #635, .T. ) ;
#1237=AXIS2_PLACEMENT_3D ( 'NONE', #552, #1528, #530 ) ;
#1239=ADVANCED_FACE ( 'NONE', ( #179 ), #1564, .T. ) ;
#1240=CARTESIAN_POINT ( 'NONE',  ( 145.0000000000000284, 2.993649167310367343, 47.64999999999998437 ) ) ;
#1241=EDGE_CURVE ( 'NONE', #473, #665, #2175, .T. ) ;
#1242=AXIS2_PLACEMENT_3D ( 'NONE', #25, #862, #419 ) ;
#1244=EDGE_LOOP ( 'NONE', ( #465, #2106, #1758, #1172 ) ) ;
#1246=CARTESIAN_POINT ( 'NONE',  ( 0.000000000000000000, 3.000000000000000000, 57.00000000000000711 ) ) ;
#1248=ORIENTED_EDGE ( 'NONE', *, *, #1383, .F. ) ;
#1249=CARTESIAN_POINT ( 'NONE',  ( 145.0000000000000284, 0.000000000000000000, -47.64999999999998437 ) ) ;
#1251=DIRECTION ( 'NONE',  ( 2.312964634635742957E-16, 0.000000000000000000, -1.000000000000000000 ) ) ;
#1255=VERTEX_POINT ( 'NONE', #1040 ) ;
#1256=FACE_OUTER_BOUND ( 'NONE', #1318, .T. ) ;
#1257=LINE ( 'NONE', #47, #418 ) ;
#1269=CARTESIAN_POINT ( 'NONE',  ( -145.0000000000000284, 2.800000000000000266, -45.00000000000000000 ) ) ;
#1270=DIRECTION ( 'NONE',  ( 0.000000000000000000, 0.000000000000000000, -1.000000000000000000 ) ) ;
#1272=EDGE_CURVE ( 'NONE', #665, #1159, #2137, .T. ) ;
#1275=CARTESIAN_POINT ( 'NONE',  ( 145.0000000000000284, 0.000000000000000000, 42.35000000000001563 ) ) ;
#1277=ORIENTED_EDGE ( 'NONE', *, *, #186, .F. ) ;
#1278=ORIENTED_EDGE ( 'NONE', *, *, #1197, .T. ) ;
#1279=AXIS2_PLACEMENT_3D ( 'NONE', #2108, #1940, #408 ) ;
#1280=DIRECTION ( 'NONE',  ( 0.000000000000000000, 0.000000000000000000, 1.000000000000000000 ) ) ;
#1286=PLANE ( 'NONE',  #714 ) ;
#1291=DIRECTION ( 'NONE',  ( 6.123233995736766036E-17, -1.000000000000000000, 0.000000000000000000 ) ) ;
#1297=FACE_BOUND ( 'NONE', #2001, .T. ) ;
#1299=ADVANCED_FACE ( 'NONE', ( #708 ), #1031, .T. ) ;
#1300=VECTOR ( 'NONE', #1720, 1000.000000000000000 ) ;
#1304=CIRCLE ( 'NONE', #177, 2.649999999999985700 ) ;
#1305=CARTESIAN_POINT ( 'NONE',  ( -145.0000000000000284, 3.000000000000001776, -42.29999999999999716 ) ) ;
#1306=ORIENTED_EDGE ( 'NONE', *, *, #1923, .F. ) ;
#1310=CARTESIAN_POINT ( 'NONE',  ( 145.0000000000000284, 3.000000000000000000, 47.64999999999998437 ) ) ;
#1314=EDGE_CURVE ( 'NONE', #1439, #353, #1257, .T. ) ;
#1315=EDGE_CURVE ( 'NONE', #1663, #1188, #997, .T. ) ;
#1316=VERTEX_POINT ( 'NONE', #1582 ) ;
#1317=DIRECTION ( 'NONE',  ( -2.312964634635742957E-16, 0.000000000000000000, 1.000000000000000000 ) ) ;
#1318=EDGE_LOOP ( 'NONE', ( #100, #695, #2130, #251 ) ) ;
#1320=CARTESIAN_POINT ( 'NONE',  ( -145.0000000000000284, 3.000000000000002665, -45.00000000000000000 ) ) ;
#1322=DIRECTION ( 'NONE',  ( 0.000000000000000000, 0.000000000000000000, -1.000000000000000000 ) ) ;
#1323=DIRECTION ( 'NONE',  ( 6.123233995736766036E-17, -1.000000000000000000, 0.000000000000000000 ) ) ;
#1326=ORIENTED_EDGE ( 'NONE', *, *, #931, .T. ) ;
#1327=DIRECTION ( 'NONE',  ( 0.000000000000000000, -1.000000000000000000, 0.000000000000000000 ) ) ;
#1328=ORIENTED_EDGE ( 'NONE', *, *, #910, .T. ) ;
#1330=FACE_OUTER_BOUND ( 'NONE', #1451, .T. ) ;
#1334=ORIENTED_EDGE ( 'NONE', *, *, #567, .T. ) ;
#1349=CARTESIAN_POINT ( 'NONE',  ( 159.9999999999999716, 10.00000000000000000, 60.00000000000001421 ) ) ;
#1352=ORIENTED_EDGE ( 'NONE', *, *, #1697, .F. ) ;
#1354=AXIS2_PLACEMENT_3D ( 'NONE', #718, #1718, #2076 ) ;
#1361=LINE ( 'NONE', #1575, #429 ) ;
#1365=AXIS2_PLACEMENT_3D ( 'NONE', #1732, #1812, #1154 ) ;
#1366=ORIENTED_EDGE ( 'NONE', *, *, #2105, .T. ) ;
#1367=DIRECTION ( 'NONE',  ( -1.000000000000000000, -6.123233995736766036E-17, -0.000000000000000000 ) ) ;
#1370=VECTOR ( 'NONE', #243, 1000.000000000000000 ) ;
#1371=ORIENTED_EDGE ( 'NONE', *, *, #645, .T. ) ;
#1377=CARTESIAN_POINT ( 'NONE',  ( 145.0000000000000284, 0.000000000000000000, 47.64999999999998437 ) ) ;
#1379=CARTESIAN_POINT ( 'NONE',  ( -157.0000000000000284, 10.00000000000000000, 57.00000000000000711 ) ) ;
#1382=EDGE_LOOP ( 'NONE', ( #1870, #332, #1278, #780 ) ) ;
#1383=EDGE_CURVE ( 'NONE', #1725, #898, #1210, .T. ) ;
#1385=FACE_OUTER_BOUND ( 'NONE', #1859, .T. ) ;
#1388=DIRECTION ( 'NONE',  ( 0.000000000000000000, 0.000000000000000000, -1.000000000000000000 ) ) ;
#1390=VERTEX_POINT ( 'NONE', #1792 ) ;
#1392=CARTESIAN_POINT ( 'NONE',  ( 145.0000000000000284, 3.000000000000000000, 45.00000000000000000 ) ) ;
#1393=CARTESIAN_POINT ( 'NONE',  ( -160.0000000000000284, 10.00000000000000000, 57.00000000000000711 ) ) ;
#1394=CARTESIAN_POINT ( 'NONE',  ( 145.0000000000000284, 2.800000000000000266, 47.70000000000000284 ) ) ;
#1395=EDGE_CURVE ( 'NONE', #353, #256, #934, .T. ) ;
#1396=ORIENTED_EDGE ( 'NONE', *, *, #1383, .T. ) ;
#1397=ADVANCED_FACE ( 'NONE', ( #82 ), #595, .F. ) ;
#1403=CARTESIAN_POINT ( 'NONE',  ( -145.0000000000000284, 2.993649167310367343, 47.64999999999998437 ) ) ;
#1405=CARTESIAN_POINT ( 'NONE',  ( -145.0000000000000284, 3.000000000000000000, 45.00000000000000000 ) ) ;
#1415=CARTESIAN_POINT ( 'NONE',  ( 145.0000000000000284, 0.000000000000000000, 45.00000000000000000 ) ) ;
#1421=VERTEX_POINT ( 'NONE', #1627 ) ;
#1422=EDGE_CURVE ( 'NONE', #694, #1700, #2145, .T. ) ;
#1423=EDGE_LOOP ( 'NONE', ( #619, #1895, #1589, #631 ) ) ;
#1424=CARTESIAN_POINT ( 'NONE',  ( -145.0000000000000284, 3.000000000000002665, 45.00000000000000000 ) ) ;
#1426=CARTESIAN_POINT ( 'NONE',  ( -160.0000000000000000, 10.00000000000000000, -59.99999999999998579 ) ) ;
#1427=DIRECTION ( 'NONE',  ( 0.000000000000000000, -0.000000000000000000, -1.000000000000000000 ) ) ;
#1434=CARTESIAN_POINT ( 'NONE',  ( 0.000000000000000000, 3.000000000000000000, 0.000000000000000000 ) ) ;
#1439=VERTEX_POINT ( 'NONE', #218 ) ;
#1442=DIRECTION ( 'NONE',  ( 0.000000000000000000, 0.000000000000000000, -1.000000000000000000 ) ) ;
#1444=VERTEX_POINT ( 'NONE', #443 ) ;
#1445=( NAMED_UNIT ( * ) SI_UNIT ( $, .STERADIAN. ) SOLID_ANGLE_UNIT ( ) );
#1447=CARTESIAN_POINT ( 'NONE',  ( 0.000000000000000000, 10.00000000000000000, 57.00000000000000711 ) ) ;
#1449=PRODUCT_CONTEXT ( 'NONE', #849, 'mechanical' ) ;
#1450=SURFACE_SIDE_STYLE ('',( #1499 ) ) ;
#1451=EDGE_LOOP ( 'NONE', ( #1127, #560, #24, #1192 ) ) ;
#1454=CARTESIAN_POINT ( 'NONE',  ( 145.0000000000000284, 0.000000000000000000, -45.00000000000000000 ) ) ;
#1458=ORIENTED_EDGE ( 'NONE', *, *, #121, .F. ) ;
#1459=DIRECTION ( 'NONE',  ( 0.000000000000000000, -1.000000000000000000, 0.000000000000000000 ) ) ;
#1460=AXIS2_PLACEMENT_3D ( 'NONE', #317, #377, #142 ) ;
#1461=CARTESIAN_POINT ( 'NONE',  ( -145.0000000000000284, 0.000000000000000000, -47.64999999999998437 ) ) ;
#1463=AXIS2_PLACEMENT_3D ( 'NONE', #2038, #658, #1151 ) ;
#1464=AXIS2_PLACEMENT_3D ( 'NONE', #1781, #252, #1280 ) ;
#1465=VERTEX_POINT ( 'NONE', #2139 ) ;
#1466=ORIENTED_EDGE ( 'NONE', *, *, #1075, .F. ) ;
#1468=ORIENTED_EDGE ( 'NONE', *, *, #1588, .F. ) ;
#1469=LINE ( 'NONE', #1911, #152 ) ;
#1472=ADVANCED_FACE ( 'NONE', ( #426, #590, #1297, #1800, #1117 ), #1286, .T. ) ;
#1473=EDGE_CURVE ( 'NONE', #898, #216, #745, .T. ) ;
#1474=LINE ( 'NONE', #1310, #1605 ) ;
#1476=( GEOMETRIC_REPRESENTATION_CONTEXT ( 3 ) GLOBAL_UNCERTAINTY_ASSIGNED_CONTEXT ( ( #1711 ) ) GLOBAL_UNIT_ASSIGNED_CONTEXT ( ( #428, #1827, #1478 ) ) REPRESENTATION_CONTEXT ( 'NONE', 'WORKASPACE' ) );
#1478=( NAMED_UNIT ( * ) SI_UNIT ( $, .STERADIAN. ) SOLID_ANGLE_UNIT ( ) );
#1482=CARTESIAN_POINT ( 'NONE',  ( 0.000000000000000000, 10.00000000000000000, 0.000000000000000000 ) ) ;
#1483=DIRECTION ( 'NONE',  ( 0.000000000000000000, 0.000000000000000000, -1.000000000000000000 ) ) ;
#1485=CARTESIAN_POINT ( 'NONE',  ( 157.0000000000000000, 10.00000000000000000, -56.99999999999999289 ) ) ;
#1488=AXIS2_PLACEMENT_3D ( 'NONE', #513, #1897, #1882 ) ;
#1490=ORIENTED_EDGE ( 'NONE', *, *, #2067, .T. ) ;
#1492=EDGE_CURVE ( 'NONE', #1531, #344, #1304, .T. ) ;
#1493=ORIENTED_EDGE ( 'NONE', *, *, #1772, .F. ) ;
#1495=DIRECTION ( 'NONE',  ( -6.123233995736766036E-17, 1.000000000000000000, -0.000000000000000000 ) ) ;
#1496=CARTESIAN_POINT ( 'NONE',  ( 145.0000000000000284, 0.000000000000000000, -45.00000000000000000 ) ) ;
#1499=SURFACE_STYLE_FILL_AREA ( #2154 ) ;
#1501=APPLICATION_CONTEXT ( 'automotive_design' ) ;
#1502=ORIENTED_EDGE ( 'NONE', *, *, #1893, .T. ) ;
#1504=DIRECTION ( 'NONE',  ( 0.000000000000000000, 0.000000000000000000, 1.000000000000000000 ) ) ;
#1510=CARTESIAN_POINT ( 'NONE',  ( -160.0000000000000000, 10.00000000000000000, -59.99999999999998579 ) ) ;
#1512=ORIENTED_EDGE ( 'NONE', *, *, #121, .T. ) ;
#1514=TOROIDAL_SURFACE ( 'NONE', #1083, 2.700000000000000622, 0.2000000000000000111 ) ;
#1519=DIRECTION ( 'NONE',  ( 1.000000000000000000, 0.000000000000000000, 0.000000000000000000 ) ) ;
#1521=LINE ( 'NONE', #1349, #250 ) ;
#1526=AXIS2_PLACEMENT_3D ( 'NONE', #2183, #326, #1519 ) ;
#1528=DIRECTION ( 'NONE',  ( 6.123233995736766036E-17, -1.000000000000000000, 0.000000000000000000 ) ) ;
#1531=VERTEX_POINT ( 'NONE', #1461 ) ;
#1534=DIRECTION ( 'NONE',  ( 0.000000000000000000, 0.000000000000000000, -1.000000000000000000 ) ) ;
#1538=DIRECTION ( 'NONE',  ( -0.000000000000000000, 1.000000000000000000, -0.000000000000000000 ) ) ;
#1540=AXIS2_PLACEMENT_3D ( 'NONE', #1482, #159, #1844 ) ;
#1544=EDGE_CURVE ( 'NONE', #835, #1255, #1106, .T. ) ;
#1545=CARTESIAN_POINT ( 'NONE',  ( -160.0000000000000000, 10.00000000000000000, -59.99999999999998579 ) ) ;
#1547=EDGE_CURVE ( 'NONE', #44, #653, #577, .T. ) ;
#1550=ORIENTED_EDGE ( 'NONE', *, *, #1568, .F. ) ;
#1554=AXIS2_PLACEMENT_3D ( 'NONE', #448, #50, #2136 ) ;
#1555=CARTESIAN_POINT ( 'NONE',  ( -160.0000000000000000, 0.000000000000000000, -59.99999999999998579 ) ) ;
#1559=ORIENTED_EDGE ( 'NONE', *, *, #1568, .T. ) ;
#1564=TOROIDAL_SURFACE ( 'NONE', #129, 2.700000000000000622, 0.2000000000000000111 ) ;
#1565=CARTESIAN_POINT ( 'NONE',  ( 145.0000000000000284, 3.000000000000000000, -42.35000000000001563 ) ) ;
#1568=EDGE_CURVE ( 'NONE', #240, #1663, #1474, .T. ) ;
#1570=VECTOR ( 'NONE', #1002, 1000.000000000000000 ) ;
#1575=CARTESIAN_POINT ( 'NONE',  ( -160.0000000000000284, 0.000000000000000000, 60.00000000000001421 ) ) ;
#1582=CARTESIAN_POINT ( 'NONE',  ( 145.0000000000000284, 3.000000000000001776, -42.29999999999999716 ) ) ;
#1586=LINE ( 'NONE', #1041, #1195 ) ;
#1588=EDGE_CURVE ( 'NONE', #216, #1670, #507, .T. ) ;
#1589=ORIENTED_EDGE ( 'NONE', *, *, #1544, .F. ) ;
#1590=ORIENTED_EDGE ( 'NONE', *, *, #1893, .F. ) ;
#1593=FACE_BOUND ( 'NONE', #1819, .T. ) ;
#1597=DIRECTION ( 'NONE',  ( -0.000000000000000000, 1.000000000000000000, -0.000000000000000000 ) ) ;
#1599=AXIS2_PLACEMENT_3D ( 'NONE', #1392, #1204, #1039 ) ;
#1600=EDGE_LOOP ( 'NONE', ( #19, #148, #35, #864 ) ) ;
#1601=ORIENTED_EDGE ( 'NONE', *, *, #1395, .F. ) ;
#1603=CARTESIAN_POINT ( 'NONE',  ( 145.0000000000000284, 2.993649167310367343, 45.00000000000000000 ) ) ;
#1605=VECTOR ( 'NONE', #2165, 1000.000000000000000 ) ;
#1606=( LENGTH_UNIT ( ) NAMED_UNIT ( * ) SI_UNIT ( .MILLI., .METRE. ) );
#1608=CARTESIAN_POINT ( 'NONE',  ( -145.0000000000000284, 0.000000000000000000, -45.00000000000000000 ) ) ;
#1615=FACE_OUTER_BOUND ( 'NONE', #843, .T. ) ;
#1627=CARTESIAN_POINT ( 'NONE',  ( -157.0000000000000000, 10.00000000000000000, -56.99999999999997868 ) ) ;
#1628=DIRECTION ( 'NONE',  ( -1.000000000000000000, 0.000000000000000000, -0.000000000000000000 ) ) ;
#1630=DIRECTION ( 'NONE',  ( -2.312964634635742957E-16, 0.000000000000000000, 1.000000000000000000 ) ) ;
#1635=CIRCLE ( 'NONE', #1526, 2.649999999999985700 ) ;
#1637=ORIENTED_EDGE ( 'NONE', *, *, #1473, .T. ) ;
#1638=CIRCLE ( 'NONE', #1960, 2.649999999999985700 ) ;
#1642=PRODUCT_DEFINITION ( 'UNKNOWN', '', #656, #1199 ) ;
#1645=CARTESIAN_POINT ( 'NONE',  ( 157.0000000000000000, 3.000000000000000000, 3.631354476378115974E-14 ) ) ;
#1646=AXIS2_PLACEMENT_3D ( 'NONE', #1656, #1323, #77 ) ;
#1656=CARTESIAN_POINT ( 'NONE',  ( 145.0000000000000284, 2.800000000000000266, 45.00000000000000000 ) ) ;
#1659=ADVANCED_FACE ( 'NONE', ( #1061 ), #1948, .T. ) ;
#1660=DIRECTION ( 'NONE',  ( 0.000000000000000000, 0.000000000000000000, 1.000000000000000000 ) ) ;
#1661=VERTEX_POINT ( 'NONE', #1933 ) ;
#1662=DIRECTION ( 'NONE',  ( 2.312964634635742957E-16, 0.000000000000000000, -1.000000000000000000 ) ) ;
#1663=VERTEX_POINT ( 'NONE', #1240 ) ;
#1666=DIRECTION ( 'NONE',  ( 6.123233995736766036E-17, -1.000000000000000000, 0.000000000000000000 ) ) ;
#1669=AXIS2_PLACEMENT_3D ( 'NONE', #1205, #26, #883 ) ;
#1670=VERTEX_POINT ( 'NONE', #202 ) ;
#1674=TOROIDAL_SURFACE ( 'NONE', #355, 2.700000000000000622, 0.2000000000000000111 ) ;
#1678=DIRECTION ( 'NONE',  ( 0.000000000000000000, 0.000000000000000000, -1.000000000000000000 ) ) ;
#1680=CIRCLE ( 'NONE', #1783, 0.1999999999999987899 ) ;
#1682=EDGE_LOOP ( 'NONE', ( #1903, #2190, #1778, #1468 ) ) ;
#1688=PLANE ( 'NONE',  #777 ) ;
#1689=ORIENTED_EDGE ( 'NONE', *, *, #819, .T. ) ;
#1690=CARTESIAN_POINT ( 'NONE',  ( 145.0000000000000284, 0.000000000000000000, 45.00000000000000000 ) ) ;
#1691=DIRECTION ( 'NONE',  ( 2.312964634635742957E-16, 0.000000000000000000, -1.000000000000000000 ) ) ;
#1693=VECTOR ( 'NONE', #770, 1000.000000000000000 ) ;
#1694=AXIS2_PLACEMENT_3D ( 'NONE', #1405, #845, #674 ) ;
#1696=EDGE_LOOP ( 'NONE', ( #337, #1087, #1076, #1203 ) ) ;
#1697=EDGE_CURVE ( 'NONE', #1316, #1670, #1070, .T. ) ;
#1700=VERTEX_POINT ( 'NONE', #120 ) ;
#1701=CARTESIAN_POINT ( 'NONE',  ( -145.0000000000000284, 2.993649167310367343, -47.64999999999998437 ) ) ;
#1704=VERTEX_POINT ( 'NONE', #1485 ) ;
#1709=DIRECTION ( 'NONE',  ( 0.000000000000000000, 0.000000000000000000, -1.000000000000000000 ) ) ;
#1711=UNCERTAINTY_MEASURE_WITH_UNIT (LENGTH_MEASURE( 1.000000000000000082E-05 ), #428, 'distance_accuracy_value', 'NONE');
#1715=ORIENTED_EDGE ( 'NONE', *, *, #580, .T. ) ;
#1716=ORIENTED_EDGE ( 'NONE', *, *, #381, .F. ) ;
#1718=DIRECTION ( 'NONE',  ( -6.123233995736766036E-17, 1.000000000000000000, -0.000000000000000000 ) ) ;
#1720=DIRECTION ( 'NONE',  ( -0.000000000000000000, 1.000000000000000000, -0.000000000000000000 ) ) ;
#1722=ADVANCED_FACE ( 'NONE', ( #276 ), #2043, .T. ) ;
#1725=VERTEX_POINT ( 'NONE', #2008 ) ;
#1726=AXIS2_PLACEMENT_3D ( 'NONE', #487, #1136, #1662 ) ;
#1727=DIRECTION ( 'NONE',  ( 0.000000000000000000, -1.000000000000000000, 0.000000000000000000 ) ) ;
#1728=DIRECTION ( 'NONE',  ( 0.000000000000000000, 0.000000000000000000, -1.000000000000000000 ) ) ;
#1731=CARTESIAN_POINT ( 'NONE',  ( -145.0000000000000284, 3.000000000000000000, -42.35000000000001563 ) ) ;
#1732=CARTESIAN_POINT ( 'NONE',  ( 145.0000000000000284, 3.000000000000002665, -45.00000000000000000 ) ) ;
#1735=VERTEX_POINT ( 'NONE', #1275 ) ;
#1736=FACE_OUTER_BOUND ( 'NONE', #1244, .T. ) ;
#1737=DIRECTION ( 'NONE',  ( -2.312964634635742957E-16, 0.000000000000000000, 1.000000000000000000 ) ) ;
#1741=LINE ( 'NONE', #392, #1878 ) ;
#1742=TOROIDAL_SURFACE ( 'NONE', #1279, 2.700000000000000622, 0.2000000000000000111 ) ;
#1746=VECTOR ( 'NONE', #603, 1000.000000000000000 ) ;
#1748=DIRECTION ( 'NONE',  ( 0.000000000000000000, 0.000000000000000000, -1.000000000000000000 ) ) ;
#1750=DIRECTION ( 'NONE',  ( 0.000000000000000000, 0.000000000000000000, -1.000000000000000000 ) ) ;
#1752=CIRCLE ( 'NONE', #103, 0.2000000000000000944 ) ;
#1755=FACE_OUTER_BOUND ( 'NONE', #214, .T. ) ;
#1758=ORIENTED_EDGE ( 'NONE', *, *, #381, .T. ) ;
#1759=DIRECTION ( 'NONE',  ( 0.000000000000000000, 0.000000000000000000, -1.000000000000000000 ) ) ;
#1762=EDGE_CURVE ( 'NONE', #833, #486, #772, .T. ) ;
#1771=PLANE ( 'NONE',  #1123 ) ;
#1772=EDGE_CURVE ( 'NONE', #833, #694, #263, .T. ) ;
#1773=DIRECTION ( 'NONE',  ( 0.000000000000000000, 0.000000000000000000, -1.000000000000000000 ) ) ;
#1778=ORIENTED_EDGE ( 'NONE', *, *, #1697, .T. ) ;
#1781=CARTESIAN_POINT ( 'NONE',  ( 145.0000000000000284, 3.000000000000000000, 45.00000000000000000 ) ) ;
#1782=DIRECTION ( 'NONE',  ( 0.000000000000000000, -0.000000000000000000, -1.000000000000000000 ) ) ;
#1783=AXIS2_PLACEMENT_3D ( 'NONE', #1394, #1190, #1534 ) ;
#1785=CARTESIAN_POINT ( 'NONE',  ( -160.0000000000000284, 10.00000000000000000, 60.00000000000001421 ) ) ;
#1788=EDGE_CURVE ( 'NONE', #1663, #1390, #1680, .T. ) ;
#1789=ORIENTED_EDGE ( 'NONE', *, *, #1145, .F. ) ;
#1790=EDGE_CURVE ( 'NONE', #415, #353, #2186, .T. ) ;
#1791=ORIENTED_EDGE ( 'NONE', *, *, #2105, .F. ) ;
#1792=CARTESIAN_POINT ( 'NONE',  ( 145.0000000000000284, 3.000000000000001776, 47.70000000000000284 ) ) ;
#1793=LINE ( 'NONE', #210, #581 ) ;
#1798=CIRCLE ( 'NONE', #1223, 2.649999999999985700 ) ;
#1800=FACE_BOUND ( 'NONE', #1864, .T. ) ;
#1807=FACE_OUTER_BOUND ( 'NONE', #1423, .T. ) ;
#1812=DIRECTION ( 'NONE',  ( -6.123233995736766036E-17, 1.000000000000000000, -0.000000000000000000 ) ) ;
#1815=ORIENTED_EDGE ( 'NONE', *, *, #1790, .F. ) ;
#1819=EDGE_LOOP ( 'NONE', ( #1111, #1352 ) ) ;
#1821=DIRECTION ( 'NONE',  ( 0.000000000000000000, 0.000000000000000000, -1.000000000000000000 ) ) ;
#1824=LINE ( 'NONE', #638, #1019 ) ;
#1826=AXIS2_PLACEMENT_3D ( 'NONE', #137, #668, #1821 ) ;
#1827=( NAMED_UNIT ( * ) PLANE_ANGLE_UNIT ( ) SI_UNIT ( $, .RADIAN. ) );
#1834=CIRCLE ( 'NONE', #875, 2.649999999999985700 ) ;
#1835=DIRECTION ( 'NONE',  ( 0.000000000000000000, -1.000000000000000000, 0.000000000000000000 ) ) ;
#1841=ORIENTED_EDGE ( 'NONE', *, *, #931, .F. ) ;
#1844=DIRECTION ( 'NONE',  ( 0.000000000000000000, -0.000000000000000000, -1.000000000000000000 ) ) ;
#1854=PLANE ( 'NONE',  #71 ) ;
#1859=EDGE_LOOP ( 'NONE', ( #606, #667, #1879, #234 ) ) ;
#1860=LINE ( 'NONE', #650, #759 ) ;
#1861=CARTESIAN_POINT ( 'NONE',  ( 159.9999999999999716, 10.00000000000000000, 60.00000000000001421 ) ) ;
#1862=CIRCLE ( 'NONE', #1460, 2.649999999999985700 ) ;
#1864=EDGE_LOOP ( 'NONE', ( #2207, #6 ) ) ;
#1867=CARTESIAN_POINT ( 'NONE',  ( -145.0000000000000284, 2.800000000000000266, 42.29999999999999716 ) ) ;
#1870=ORIENTED_EDGE ( 'NONE', *, *, #929, .T. ) ;
#1877=EDGE_CURVE ( 'NONE', #1255, #848, #2077, .T. ) ;
#1878=VECTOR ( 'NONE', #350, 1000.000000000000000 ) ;
#1879=ORIENTED_EDGE ( 'NONE', *, *, #1272, .T. ) ;
#1882=DIRECTION ( 'NONE',  ( 0.000000000000000000, -1.000000000000000000, 0.000000000000000000 ) ) ;
#1884=LINE ( 'NONE', #1565, #1300 ) ;
#1889=CARTESIAN_POINT ( 'NONE',  ( 145.0000000000000284, 2.800000000000000266, 45.00000000000000000 ) ) ;
#1891=DIRECTION ( 'NONE',  ( -0.000000000000000000, 1.000000000000000000, -0.000000000000000000 ) ) ;
#1893=EDGE_CURVE ( 'NONE', #848, #415, #1361, .T. ) ;
#1895=ORIENTED_EDGE ( 'NONE', *, *, #1877, .F. ) ;
#1897=DIRECTION ( 'NONE',  ( -1.000000000000000000, -6.123233995736766036E-17, -0.000000000000000000 ) ) ;
#1898=EDGE_CURVE ( 'NONE', #1704, #1421, #1908, .T. ) ;
#1900=EDGE_CURVE ( 'NONE', #344, #1531, #1862, .T. ) ;
#1903=ORIENTED_EDGE ( 'NONE', *, *, #509, .T. ) ;
#1906=DIRECTION ( 'NONE',  ( 0.000000000000000000, 0.000000000000000000, -1.000000000000000000 ) ) ;
#1907=LINE ( 'NONE', #170, #88 ) ;
#1908=LINE ( 'NONE', #2021, #1570 ) ;
#1911=CARTESIAN_POINT ( 'NONE',  ( 156.9999999999999716, 10.00000000000000000, 57.00000000000000711 ) ) ;
#1915=ORIENTED_EDGE ( 'NONE', *, *, #482, .F. ) ;
#1916=LINE ( 'NONE', #882, #461 ) ;
#1921=CARTESIAN_POINT ( 'NONE',  ( 156.9999999999999716, 10.00000000000000000, 57.00000000000000711 ) ) ;
#1923=EDGE_CURVE ( 'NONE', #1661, #1439, #199, .T. ) ;
#1924=EDGE_LOOP ( 'NONE', ( #751, #1334, #1559, #2064 ) ) ;
#1928=FACE_BOUND ( 'NONE', #2047, .T. ) ;
#1931=DIRECTION ( 'NONE',  ( 6.123233995736766036E-17, -1.000000000000000000, 0.000000000000000000 ) ) ;
#1933=CARTESIAN_POINT ( 'NONE',  ( 159.9999999999999716, 10.00000000000000000, 60.00000000000001421 ) ) ;
#1934=ADVANCED_FACE ( 'NONE', ( #154 ), #27, .F. ) ;
#1937=ADVANCED_FACE ( 'NONE', ( #1943, #913, #1113, #1928, #1593 ), #48, .F. ) ;
#1938=CIRCLE ( 'NONE', #67, 2.649999999999985700 ) ;
#1940=DIRECTION ( 'NONE',  ( 6.123233995736766036E-17, -1.000000000000000000, 0.000000000000000000 ) ) ;
#1942=DIRECTION ( 'NONE',  ( 0.000000000000000000, 0.000000000000000000, -1.000000000000000000 ) ) ;
#1943=FACE_OUTER_BOUND ( 'NONE', #1382, .T. ) ;
#1945=CIRCLE ( 'NONE', #986, 0.1999999999999987899 ) ;
#1946=LINE ( 'NONE', #412, #517 ) ;
#1948=PLANE ( 'NONE',  #437 ) ;
#1951=DIRECTION ( 'NONE',  ( 0.000000000000000000, 0.000000000000000000, -1.000000000000000000 ) ) ;
#1955=AXIS2_PLACEMENT_3D ( 'NONE', #1393, #1942, #69 ) ;
#1959=ADVANCED_FACE ( 'NONE', ( #238 ), #390, .F. ) ;
#1960=AXIS2_PLACEMENT_3D ( 'NONE', #1415, #697, #1748 ) ;
#1962=PRODUCT ( 'tray', 'tray', '', ( #1449 ) ) ;
#1963=VERTEX_POINT ( 'NONE', #574 ) ;
#1970=EDGE_CURVE ( 'NONE', #835, #256, #1793, .T. ) ;
#1971=CARTESIAN_POINT ( 'NONE',  ( -145.0000000000000284, 2.800000000000000266, 47.70000000000000284 ) ) ;
#1972=DIRECTION ( 'NONE',  ( -2.312964634635742957E-16, -0.000000000000000000, 1.000000000000000000 ) ) ;
#1976=ORIENTED_EDGE ( 'NONE', *, *, #1422, .F. ) ;
#1977=DIRECTION ( 'NONE',  ( 1.000000000000000000, 0.000000000000000000, 0.000000000000000000 ) ) ;
#1982=FACE_OUTER_BOUND ( 'NONE', #417, .T. ) ;
#1983=AXIS2_PLACEMENT_3D ( 'NONE', #73, #936, #768 ) ;
#1985=VECTOR ( 'NONE', #1327, 1000.000000000000000 ) ;
#1989=ORIENTED_EDGE ( 'NONE', *, *, #1473, .F. ) ;
#2001=EDGE_LOOP ( 'NONE', ( #1248, #716 ) ) ;
#2004=ORIENTED_EDGE ( 'NONE', *, *, #1788, .T. ) ;
#2008=CARTESIAN_POINT ( 'NONE',  ( 145.0000000000000284, 0.000000000000000000, -42.35000000000001563 ) ) ;
#2011=ADVANCED_FACE ( 'NONE', ( #1615 ), #726, .T. ) ;
#2013=CARTESIAN_POINT ( 'NONE',  ( 156.9999999999999716, 10.00000000000000000, 60.00000000000001421 ) ) ;
#2014=EDGE_LOOP ( 'NONE', ( #235, #308 ) ) ;
#2016=FACE_BOUND ( 'NONE', #802, .T. ) ;
#2019=ORIENTED_EDGE ( 'NONE', *, *, #1900, .F. ) ;
#2020=DIRECTION ( 'NONE',  ( 0.000000000000000000, 0.000000000000000000, -1.000000000000000000 ) ) ;
#2021=CARTESIAN_POINT ( 'NONE',  ( -2.471980953266949321E-15, 10.00000000000000000, -56.99999999999998579 ) ) ;
#2025=EDGE_LOOP ( 'NONE', ( #1815, #1590, #1144, #1601 ) ) ;
#2028=ORIENTED_EDGE ( 'NONE', *, *, #467, .F. ) ;
#2033=ORIENTED_EDGE ( 'NONE', *, *, #1877, .T. ) ;
#2038=CARTESIAN_POINT ( 'NONE',  ( -145.0000000000000284, 2.993649167310367343, 45.00000000000000000 ) ) ;
#2040=ORIENTED_EDGE ( 'NONE', *, *, #1241, .F. ) ;
#2042=CARTESIAN_POINT ( 'NONE',  ( 159.9999999999999716, 0.000000000000000000, 60.00000000000001421 ) ) ;
#2043=TOROIDAL_SURFACE ( 'NONE', #1646, 2.700000000000000622, 0.2000000000000000111 ) ;
#2046=CIRCLE ( 'NONE', #1826, 2.700000000000001066 ) ;
#2047=EDGE_LOOP ( 'NONE', ( #178, #1086 ) ) ;
#2048=VECTOR ( 'NONE', #1977, 1000.000000000000000 ) ;
#2049=ORIENTED_EDGE ( 'NONE', *, *, #266, .T. ) ;
#2056=CIRCLE ( 'NONE', #182, 0.1999999999999987899 ) ;
#2064=ORIENTED_EDGE ( 'NONE', *, *, #1092, .F. ) ;
#2067=EDGE_CURVE ( 'NONE', #60, #396, #659, .T. ) ;
#2075=CARTESIAN_POINT ( 'NONE',  ( 145.0000000000000284, 3.000000000000000000, -45.00000000000000000 ) ) ;
#2076=DIRECTION ( 'NONE',  ( 0.000000000000000000, 0.000000000000000000, -1.000000000000000000 ) ) ;
#2077=LINE ( 'NONE', #494, #712 ) ;
#2079=ORIENTED_EDGE ( 'NONE', *, *, #1092, .T. ) ;
#2080=CARTESIAN_POINT ( 'NONE',  ( -145.0000000000000284, 2.800000000000000266, -42.29999999999999716 ) ) ;
#2084=AXIS2_PLACEMENT_3D ( 'NONE', #865, #904, #1227 ) ;
#2087=AXIS2_PLACEMENT_3D ( 'NONE', #253, #39, #1442 ) ;
#2088=EDGE_LOOP ( 'NONE', ( #1046, #1689, #2040, #1716 ) ) ;
#2090=LINE ( 'NONE', #1048, #527 ) ;
#2093=ADVANCED_FACE ( 'NONE', ( #732 ), #1771, .F. ) ;
#2094=CARTESIAN_POINT ( 'NONE',  ( -145.0000000000000284, 3.000000000000001776, 47.70000000000000284 ) ) ;
#2096=ORIENTED_EDGE ( 'NONE', *, *, #744, .F. ) ;
#2104=DIRECTION ( 'NONE',  ( 0.000000000000000000, -1.000000000000000000, 0.000000000000000000 ) ) ;
#2105=EDGE_CURVE ( 'NONE', #1704, #44, #70, .T. ) ;
#2106=ORIENTED_EDGE ( 'NONE', *, *, #1492, .T. ) ;
#2108=CARTESIAN_POINT ( 'NONE',  ( -145.0000000000000284, 2.800000000000000266, 45.00000000000000000 ) ) ;
#2111=CLOSED_SHELL ( 'NONE', ( #1722, #946, #352, #345, #2204, #1934, #1214, #146, #1397, #287, #941, #305, #1937, #66, #423, #1959, #2129, #2093, #1472, #2173, #1107, #1659, #1299, #246, #2011, #171, #1239 ) ) ;
#2113=VECTOR ( 'NONE', #1597, 1000.000000000000000 ) ;
#2116=CIRCLE ( 'NONE', #2084, 2.649999999999985700 ) ;
#2120=DIRECTION ( 'NONE',  ( 0.000000000000000000, -1.000000000000000000, 0.000000000000000000 ) ) ;
#2121=AXIS2_PLACEMENT_3D ( 'NONE', #1090, #902, #434 ) ;
#2125=DIRECTION ( 'NONE',  ( 1.000000000000000000, 6.123233995736766036E-17, -1.224646799147353207E-16 ) ) ;
#2129=ADVANCED_FACE ( 'NONE', ( #1807 ), #109, .F. ) ;
#2130=ORIENTED_EDGE ( 'NONE', *, *, #1236, .T. ) ;
#2131=CARTESIAN_POINT ( 'NONE',  ( -160.0000000000000000, 0.000000000000000000, -59.99999999999998579 ) ) ;
#2132=CARTESIAN_POINT ( 'NONE',  ( 156.9999999999999432, 10.00000000000000000, -56.99999999999999289 ) ) ;
#2136=DIRECTION ( 'NONE',  ( 0.000000000000000000, 0.000000000000000000, 1.000000000000000000 ) ) ;
#2137=CIRCLE ( 'NONE', #1488, 0.2000000000000000944 ) ;
#2138=ADVANCED_BREP_SHAPE_REPRESENTATION ( '', ( #969, #30 ), #1049 ) ;
#2139=CARTESIAN_POINT ( 'NONE',  ( -145.0000000000000284, 0.000000000000000000, 47.64999999999998437 ) ) ;
#2145=LINE ( 'NONE', #1246, #2048 ) ;
#2147=ORIENTED_EDGE ( 'NONE', *, *, #334, .F. ) ;
#2154=FILL_AREA_STYLE ('',( #131 ) ) ;
#2155=ORIENTED_EDGE ( 'NONE', *, *, #734, .T. ) ;
#2159=CARTESIAN_POINT ( 'NONE',  ( 159.9999999999999716, 10.00000000000000000, 60.00000000000001421 ) ) ;
#2161=AXIS2_PLACEMENT_3D ( 'NONE', #1146, #323, #1504 ) ;
#2163=AXIS2_PLACEMENT_3D ( 'NONE', #1971, #2125, #613 ) ;
#2165=DIRECTION ( 'NONE',  ( -0.000000000000000000, 1.000000000000000000, -0.000000000000000000 ) ) ;
#2167=SURFACE_STYLE_USAGE ( .BOTH. , #1450 ) ;
#2169=FACE_OUTER_BOUND ( 'NONE', #2088, .T. ) ;
#2170=ORIENTED_EDGE ( 'NONE', *, *, #334, .T. ) ;
#2173=ADVANCED_FACE ( 'NONE', ( #654 ), #1854, .T. ) ;
#2174=CARTESIAN_POINT ( 'NONE',  ( 145.0000000000000284, 3.000000000000002665, 45.00000000000000000 ) ) ;
#2175=CIRCLE ( 'NONE', #1237, 2.649999999999985700 ) ;
#2181=EDGE_LOOP ( 'NONE', ( #2019, #225 ) ) ;
#2183=CARTESIAN_POINT ( 'NONE',  ( 145.0000000000000284, 2.993649167310367343, 45.00000000000000000 ) ) ;
#2186=LINE ( 'NONE', #2042, #501 ) ;
#2188=PRESENTATION_STYLE_ASSIGNMENT (( #2167 ) ) ;
#2190=ORIENTED_EDGE ( 'NONE', *, *, #2208, .T. ) ;
#2193=CYLINDRICAL_SURFACE ( 'NONE', #1599, 2.649999999999985700 ) ;
#2198=ORIENTED_EDGE ( 'NONE', *, *, #1898, .F. ) ;
#2199=VECTOR ( 'NONE', #886, 1000.000000000000000 ) ;
#2202=CIRCLE ( 'NONE', #2163, 0.1999999999999987899 ) ;
#2204=ADVANCED_FACE ( 'NONE', ( #2169 ), #826, .F. ) ;
#2207=ORIENTED_EDGE ( 'NONE', *, *, #281, .F. ) ;
#2208=EDGE_CURVE ( 'NONE', #1444, #1316, #2056, .T. ) ;
#2217=ORIENTED_EDGE ( 'NONE', *, *, #767, .T. ) ;
#2218=VERTEX_POINT ( 'NONE', #1305 ) ;
#2219=AXIS2_PLACEMENT_3D ( 'NONE', #529, #1727, #1709 ) ;
#2223=CARTESIAN_POINT ( 'NONE',  ( -157.0000000000000000, 3.000000000000000000, -56.99999999999997868 ) ) ;
#2226=CARTESIAN_POINT ( 'NONE',  ( -145.0000000000000284, 0.000000000000000000, 45.00000000000000000 ) ) ;
#2241=COLOUR_RGB('Light Blue',0.38,0.62,0.78);
#2242=FILL_AREA_STYLE_COLOUR('',#2241);
#2243=FILL_AREA_STYLE('',(#2242));
#2244=SURFACE_STYLE_FILL_AREA(#2243);
#2245=SURFACE_SIDE_STYLE('',(#2244));
#2246=SURFACE_STYLE_USAGE(.BOTH.,#2245);
#2247=PRESENTATION_STYLE_ASSIGNMENT((#2246));
ENDSEC;
END-ISO-10303-21;
